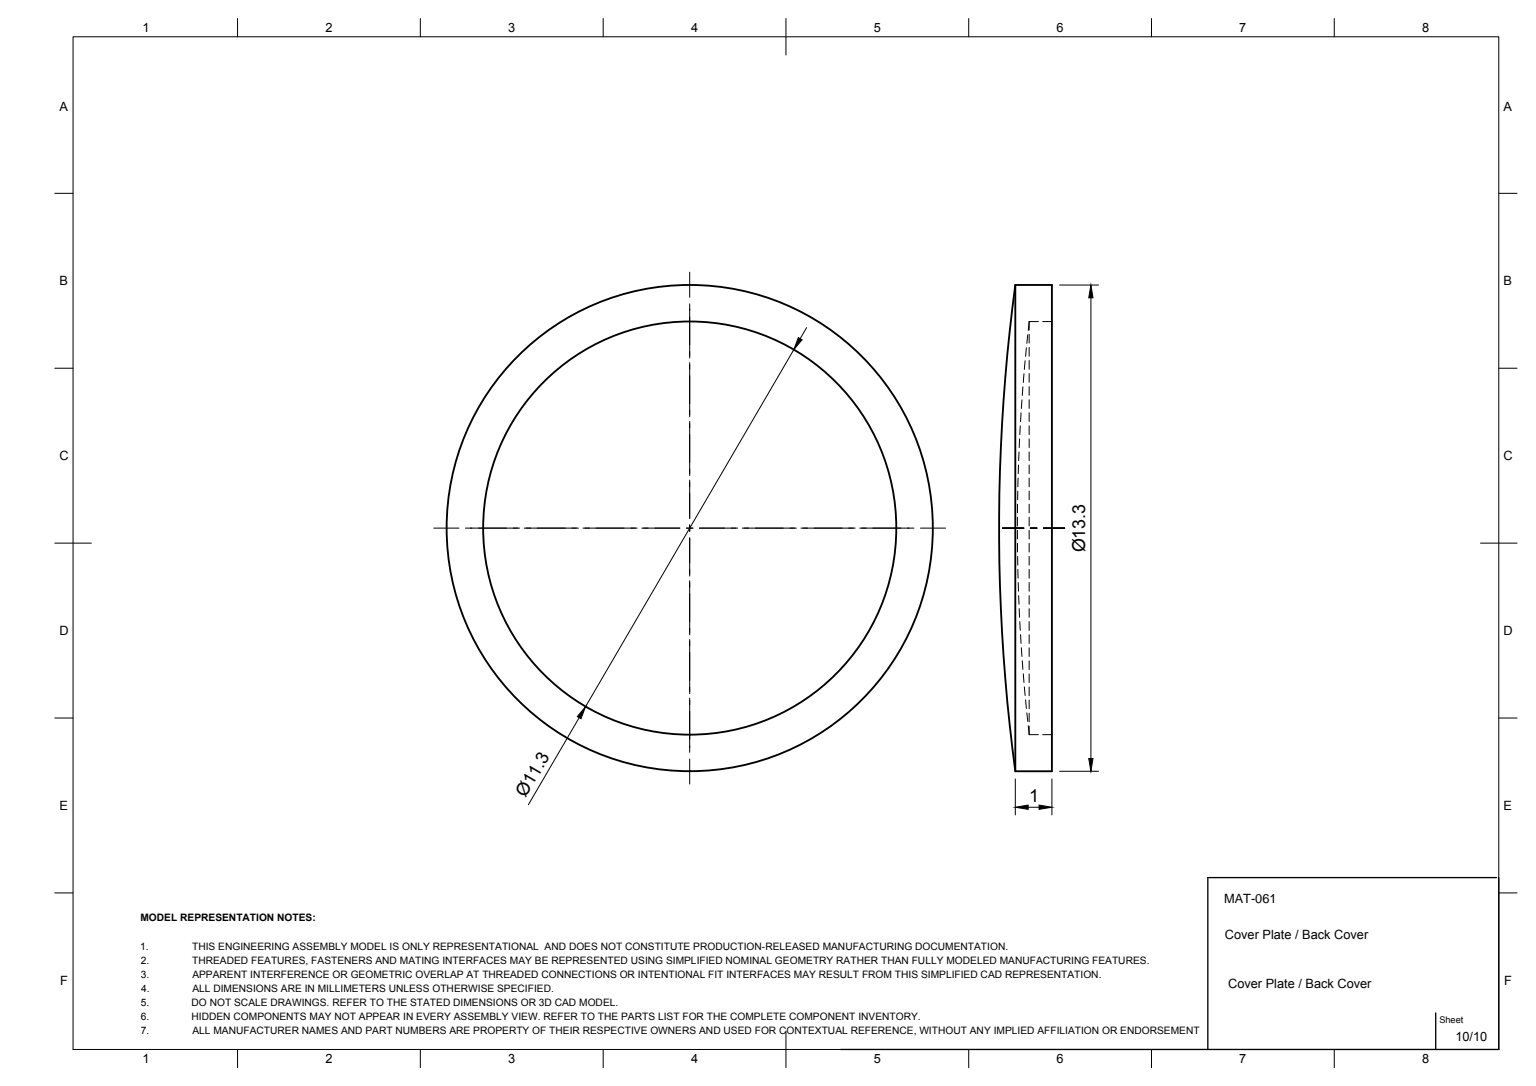
ISO-10303-21;
HEADER;
/* Generated by software containing ST-Developer
 * from STEP Tools, Inc. (www.steptools.com) 
 */

FILE_DESCRIPTION(
/* description */ ('', 'CAx-IF Rec.Pracs.---Representation and Presentation of Product Manufa
cturing Information (PMI)---4.0---2014-10-13'),
/* implementation_level */ '2;1');

FILE_NAME(
/* name */ 'Cover Plate _ Back Cover.step',
/* time_stamp */ '2026-10-28T14:45:12+01:00',
/* author */ (''),
/* organization */ (''),
/* preprocessor_version */ 'ST-DEVELOPER v20.2',
/* originating_system */ 'Autodesk Translation Framework v15.17.0.0',
/* authorisation */ '');

FILE_SCHEMA (('AP242_MANAGED_MODEL_BASED_3D_ENGINEERING_MIM_LF { 1 0 10303 442 2 1 4 }'));
ENDSEC;

DATA;
#10=MECHANICAL_DESIGN_GEOMETRIC_PRESENTATION_REPRESENTATION('',(#270),#52164);
#244=SHAPE_REPRESENTATION_RELATIONSHIP('SRR','None',#52223,#257);
#257=ADVANCED_BREP_SHAPE_REPRESENTATION('',(#283),#52163);
#270=STYLED_ITEM('',(#52332),#283);
#283=MANIFOLD_SOLID_BREP('Body1',#9130);
#286=SPHERICAL_SURFACE('',#10190,50.);
#287=SPHERICAL_SURFACE('',#10195,49.5);
#322=FACE_BOUND('',#1622,.T.);
#517=PLANE('',#10185);
#1050=FACE_OUTER_BOUND('',#1621,.T.);
#1051=FACE_OUTER_BOUND('',#1623,.T.);
#1052=FACE_OUTER_BOUND('',#1624,.T.);
#1053=FACE_OUTER_BOUND('',#1625,.T.);
#1054=FACE_OUTER_BOUND('',#1626,.T.);
#1621=EDGE_LOOP('',(#8330));
#1622=EDGE_LOOP('',(#8331));
#1623=EDGE_LOOP('',(#8332,#8333,#8334,#8335));
#1624=EDGE_LOOP('',(#8336,#8337,#8338));
#1625=EDGE_LOOP('',(#8339,#8340,#8341,#8342,#8343));
#1626=EDGE_LOOP('',(#8344,#8345,#8346,#8347));
#2087=CIRCLE('',#10186,6.65);
#2088=CIRCLE('',#10187,5.65);
#2089=CIRCLE('',#10189,6.65);
#2090=CIRCLE('',#10191,50.);
#2091=CIRCLE('',#10193,5.65);
#2092=CIRCLE('',#10194,5.65);
#2093=CIRCLE('',#10196,49.5);
#2925=LINE('',#52108,#3390);
#2926=LINE('',#52117,#3391);
#3390=VECTOR('',#12501,6.65);
#3391=VECTOR('',#12512,5.65);
#4249=VERTEX_POINT('',#52102);
#4250=VERTEX_POINT('',#52104);
#4251=VERTEX_POINT('',#52107);
#4252=VERTEX_POINT('',#52111);
#4253=VERTEX_POINT('',#52114);
#4254=VERTEX_POINT('',#52115);
#4255=VERTEX_POINT('',#52120);
#5611=EDGE_CURVE('',#4249,#4249,#2087,.T.);
#5612=EDGE_CURVE('',#4250,#4250,#2088,.T.);
#5613=EDGE_CURVE('',#4249,#4251,#2925,.T.);
#5614=EDGE_CURVE('',#4251,#4251,#2089,.T.);
#5615=EDGE_CURVE('',#4251,#4252,#2090,.T.);
#5616=EDGE_CURVE('',#4253,#4254,#2091,.T.);
#5617=EDGE_CURVE('',#4253,#4250,#2926,.T.);
#5618=EDGE_CURVE('',#4254,#4253,#2092,.T.);
#5619=EDGE_CURVE('',#4255,#4254,#2093,.T.);
#8330=ORIENTED_EDGE('',*,*,#5611,.T.);
#8331=ORIENTED_EDGE('',*,*,#5612,.F.);
#8332=ORIENTED_EDGE('',*,*,#5611,.F.);
#8333=ORIENTED_EDGE('',*,*,#5613,.T.);
#8334=ORIENTED_EDGE('',*,*,#5614,.T.);
#8335=ORIENTED_EDGE('',*,*,#5613,.F.);
#8336=ORIENTED_EDGE('',*,*,#5614,.F.);
#8337=ORIENTED_EDGE('',*,*,#5615,.T.);
#8338=ORIENTED_EDGE('',*,*,#5615,.F.);
#8339=ORIENTED_EDGE('',*,*,#5616,.F.);
#8340=ORIENTED_EDGE('',*,*,#5617,.T.);
#8341=ORIENTED_EDGE('',*,*,#5612,.T.);
#8342=ORIENTED_EDGE('',*,*,#5617,.F.);
#8343=ORIENTED_EDGE('',*,*,#5618,.F.);
#8344=ORIENTED_EDGE('',*,*,#5616,.T.);
#8345=ORIENTED_EDGE('',*,*,#5619,.F.);
#8346=ORIENTED_EDGE('',*,*,#5619,.T.);
#8347=ORIENTED_EDGE('',*,*,#5618,.T.);
#8579=CYLINDRICAL_SURFACE('',#10188,6.65);
#8580=CYLINDRICAL_SURFACE('',#10192,5.65);
#9113=ADVANCED_FACE('',(#1050,#322),#517,.T.);
#9114=ADVANCED_FACE('',(#1051),#8579,.T.);
#9115=ADVANCED_FACE('',(#1052),#286,.T.);
#9116=ADVANCED_FACE('',(#1053),#8580,.F.);
#9117=ADVANCED_FACE('',(#1054),#287,.F.);
#9130=CLOSED_SHELL('',(#9113,#9114,#9115,#9116,#9117));
#10184=AXIS2_PLACEMENT_3D('',#52100,#12491,#12492);
#10185=AXIS2_PLACEMENT_3D('',#52101,#12493,#12494);
#10186=AXIS2_PLACEMENT_3D('',#52103,#12495,#12496);
#10187=AXIS2_PLACEMENT_3D('',#52105,#12497,#12498);
#10188=AXIS2_PLACEMENT_3D('',#52106,#12499,#12500);
#10189=AXIS2_PLACEMENT_3D('',#52109,#12502,#12503);
#10190=AXIS2_PLACEMENT_3D('',#52110,#12504,#12505);
#10191=AXIS2_PLACEMENT_3D('',#52112,#12506,#12507);
#10192=AXIS2_PLACEMENT_3D('',#52113,#12508,#12509);
#10193=AXIS2_PLACEMENT_3D('',#52116,#12510,#12511);
#10194=AXIS2_PLACEMENT_3D('',#52118,#12513,#12514);
#10195=AXIS2_PLACEMENT_3D('',#52119,#12515,#12516);
#10196=AXIS2_PLACEMENT_3D('',#52121,#12517,#12518);
#12491=DIRECTION('axis',(0.,0.,1.));
#12492=DIRECTION('refdir',(1.,0.,0.));
#12493=DIRECTION('center_axis',(0.,0.,1.));
#12494=DIRECTION('ref_axis',(0.,1.,0.));
#12495=DIRECTION('center_axis',(0.,0.,1.));
#12496=DIRECTION('ref_axis',(0.,-1.,0.));
#12497=DIRECTION('center_axis',(0.,0.,1.));
#12498=DIRECTION('ref_axis',(0.,-1.,0.));
#12499=DIRECTION('center_axis',(0.,0.,1.));
#12500=DIRECTION('ref_axis',(0.,1.,0.));
#12501=DIRECTION('',(0.,0.,-1.));
#12502=DIRECTION('center_axis',(0.,0.,1.));
#12503=DIRECTION('ref_axis',(0.,-1.,0.));
#12504=DIRECTION('center_axis',(0.,6.12323399573676E-17,1.));
#12505=DIRECTION('ref_axis',(0.,1.,0.));
#12506=DIRECTION('center_axis',(1.,1.22464679914735E-16,0.));
#12507=DIRECTION('ref_axis',(1.22464679914735E-16,-1.,0.));
#12508=DIRECTION('center_axis',(0.,0.,1.));
#12509=DIRECTION('ref_axis',(0.,-1.,0.));
#12510=DIRECTION('center_axis',(0.,0.,1.));
#12511=DIRECTION('ref_axis',(0.,-1.,0.));
#12512=DIRECTION('',(0.,0.,1.));
#12513=DIRECTION('center_axis',(0.,0.,1.));
#12514=DIRECTION('ref_axis',(0.,-1.,0.));
#12515=DIRECTION('center_axis',(0.,6.12323399573676E-17,1.));
#12516=DIRECTION('ref_axis',(0.,1.,0.));
#12517=DIRECTION('center_axis',(-1.,-1.22464679914735E-16,0.));
#12518=DIRECTION('ref_axis',(1.22464679914735E-16,-1.,0.));
#52100=CARTESIAN_POINT('',(0.,0.,0.));
#52101=CARTESIAN_POINT('Origin',(0.,0.,0.));
#52102=CARTESIAN_POINT('',(8.1439012143299E-16,-6.65,0.));
#52103=CARTESIAN_POINT('Origin',(0.,0.,0.));
#52104=CARTESIAN_POINT('',(0.,5.65,0.));
#52105=CARTESIAN_POINT('Origin',(0.,0.,0.));
#52106=CARTESIAN_POINT('Origin',(0.,0.,-1.51640802568));
#52107=CARTESIAN_POINT('',(8.1439012143299E-16,-6.65,-1.));
#52108=CARTESIAN_POINT('',(8.1439012143299E-16,-6.65,-1.51640802568));
#52109=CARTESIAN_POINT('Origin',(0.,0.,-1.));
#52110=CARTESIAN_POINT('Origin',(0.,0.,48.5558018803));
#52111=CARTESIAN_POINT('',(3.74939945665464E-31,-3.06161699786838E-15,-1.4441981197));
#52112=CARTESIAN_POINT('Origin',(0.,0.,48.5558018803));
#52113=CARTESIAN_POINT('Origin',(0.,0.,0.));
#52114=CARTESIAN_POINT('',(0.,5.65,-0.6206914879705));
#52115=CARTESIAN_POINT('',(6.91925441518255E-16,-5.65,-0.620691487970504));
#52116=CARTESIAN_POINT('Origin',(0.,0.,-0.6206914879705));
#52117=CARTESIAN_POINT('',(-6.91925441518255E-16,5.65,0.));
#52118=CARTESIAN_POINT('Origin',(0.,0.,-0.6206914879705));
#52119=CARTESIAN_POINT('Origin',(0.,0.,48.5558018803));
#52120=CARTESIAN_POINT('',(3.7119054620881E-31,-3.0310008278897E-15,-0.944198119699999));
#52121=CARTESIAN_POINT('Origin',(0.,0.,48.5558018803));
#52148=UNCERTAINTY_MEASURE_WITH_UNIT(LENGTH_MEASURE(0.01),#52165,
'DISTANCE_ACCURACY_VALUE',
'Maximum model space distance between geometric entities at asserted c
onnectivities');
#52149=UNCERTAINTY_MEASURE_WITH_UNIT(LENGTH_MEASURE(0.01),#52165,
'DISTANCE_ACCURACY_VALUE',
'Maximum model space distance between geometric entities at asserted c
onnectivities');
#52163=(
GEOMETRIC_REPRESENTATION_CONTEXT(3)
GLOBAL_UNCERTAINTY_ASSIGNED_CONTEXT((#52148))
GLOBAL_UNIT_ASSIGNED_CONTEXT((#52165,#52167,#52168))
REPRESENTATION_CONTEXT('','3D')
);
#52164=(
GEOMETRIC_REPRESENTATION_CONTEXT(3)
GLOBAL_UNCERTAINTY_ASSIGNED_CONTEXT((#52149))
GLOBAL_UNIT_ASSIGNED_CONTEXT((#52165,#52167,#52168))
REPRESENTATION_CONTEXT('','3D')
);
#52165=(
LENGTH_UNIT()
NAMED_UNIT(*)
SI_UNIT(.MILLI.,.METRE.)
);
#52167=(
NAMED_UNIT(*)
PLANE_ANGLE_UNIT()
SI_UNIT($,.RADIAN.)
);
#52168=(
NAMED_UNIT(*)
SI_UNIT($,.STERADIAN.)
SOLID_ANGLE_UNIT()
);
#52182=SHAPE_DEFINITION_REPRESENTATION(#52196,#52223);
#52196=PRODUCT_DEFINITION_SHAPE('',$,#52238);
#52223=SHAPE_REPRESENTATION('',(#10184),#52163);
#52224=PRODUCT_DEFINITION_CONTEXT('part definition',#52268,'design');
#52238=PRODUCT_DEFINITION('Cover Plate / Back Cover',
'Cover Plate / Back Cover',#52252,#52224);
#52252=PRODUCT_DEFINITION_FORMATION('',$,#52283);
#52268=APPLICATION_CONTEXT('Managed model based 3d engineering');
#52269=PRODUCT_CONTEXT('part definition',#52268,'mechanical');
#52283=PRODUCT('Cover Plate / Back Cover','Cover Plate / Back Cover',
'NOT SPECIFIED',(#52269));
#52326=COLOUR_RGB('Off White',0.89,0.88,0.83);
#52327=FILL_AREA_STYLE_COLOUR('',#52326);
#52328=FILL_AREA_STYLE('',(#52327));
#52329=SURFACE_STYLE_FILL_AREA(#52328);
#52330=SURFACE_SIDE_STYLE('',(#52329));
#52331=SURFACE_STYLE_USAGE(.BOTH.,#52330);
#52332=PRESENTATION_STYLE_ASSIGNMENT((#52331));
ENDSEC;
END-ISO-10303-21;
